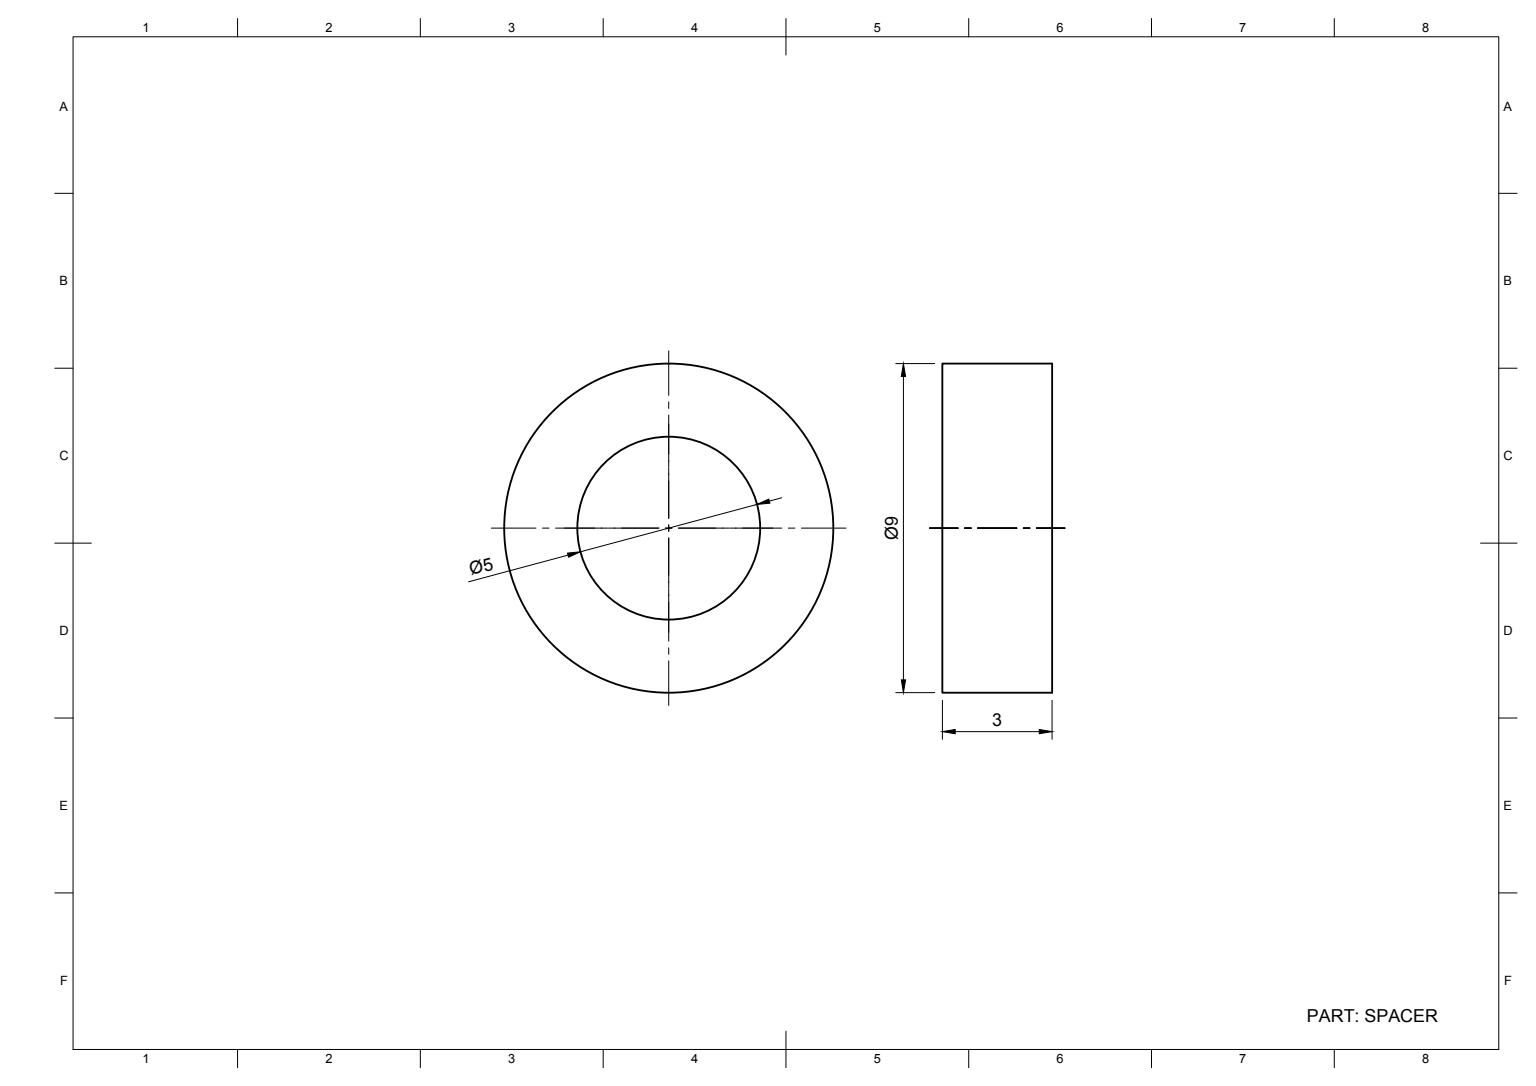
ISO-10303-21;
HEADER;
/* Generated by software containing ST-Developer
 * from STEP Tools, Inc. (www.steptools.com) 
 */

FILE_DESCRIPTION(
/* description */ (''),
/* implementation_level */ '2;1');

FILE_NAME(
/* name */ 'Spacer.step',
/* time_stamp */ '2026-09-20T21:52:48+06:00',
/* author */ (''),
/* organization */ (''),
/* preprocessor_version */ 'ST-DEVELOPER v20.2',
/* originating_system */ 'Autodesk Translation Framework v15.15.0.0',
/* authorisation */ '');

FILE_SCHEMA (('AUTOMOTIVE_DESIGN { 1 0 10303 214 3 1 1 }'));
ENDSEC;

DATA;
#10=MECHANICAL_DESIGN_GEOMETRIC_PRESENTATION_REPRESENTATION('',(#66),#2203);
#50=SHAPE_REPRESENTATION_RELATIONSHIP('SRR','None',#2242,#58);
#58=ADVANCED_BREP_SHAPE_REPRESENTATION('',(#74),#2202);
#66=STYLED_ITEM('',(#2286),#74);
#74=MANIFOLD_SOLID_BREP('Spacer',#1233);
#87=FACE_BOUND('',#308,.T.);
#88=FACE_BOUND('',#312,.T.);
#133=CIRCLE('',#1442,4.5);
#134=CIRCLE('',#1443,2.5);
#135=CIRCLE('',#1445,4.5);
#136=CIRCLE('',#1447,2.5);
#159=CYLINDRICAL_SURFACE('',#1444,4.5);
#160=CYLINDRICAL_SURFACE('',#1446,2.5);
#226=FACE_OUTER_BOUND('',#307,.T.);
#227=FACE_OUTER_BOUND('',#309,.T.);
#228=FACE_OUTER_BOUND('',#310,.T.);
#229=FACE_OUTER_BOUND('',#311,.T.);
#307=EDGE_LOOP('',(#1100));
#308=EDGE_LOOP('',(#1101));
#309=EDGE_LOOP('',(#1102,#1103,#1104,#1105));
#310=EDGE_LOOP('',(#1106,#1107,#1108,#1109));
#311=EDGE_LOOP('',(#1110));
#312=EDGE_LOOP('',(#1111));
#421=LINE('',#2169,#531);
#422=LINE('',#2174,#532);
#531=VECTOR('',#1809,4.5);
#532=VECTOR('',#1816,2.5);
#634=VERTEX_POINT('',#2163);
#635=VERTEX_POINT('',#2165);
#636=VERTEX_POINT('',#2168);
#637=VERTEX_POINT('',#2172);
#790=EDGE_CURVE('',#634,#634,#133,.T.);
#791=EDGE_CURVE('',#635,#635,#134,.T.);
#792=EDGE_CURVE('',#634,#636,#421,.T.);
#793=EDGE_CURVE('',#636,#636,#135,.T.);
#794=EDGE_CURVE('',#637,#637,#136,.T.);
#795=EDGE_CURVE('',#637,#635,#422,.T.);
#1100=ORIENTED_EDGE('',*,*,#790,.T.);
#1101=ORIENTED_EDGE('',*,*,#791,.T.);
#1102=ORIENTED_EDGE('',*,*,#790,.F.);
#1103=ORIENTED_EDGE('',*,*,#792,.T.);
#1104=ORIENTED_EDGE('',*,*,#793,.F.);
#1105=ORIENTED_EDGE('',*,*,#792,.F.);
#1106=ORIENTED_EDGE('',*,*,#794,.F.);
#1107=ORIENTED_EDGE('',*,*,#795,.T.);
#1108=ORIENTED_EDGE('',*,*,#791,.F.);
#1109=ORIENTED_EDGE('',*,*,#795,.F.);
#1110=ORIENTED_EDGE('',*,*,#793,.T.);
#1111=ORIENTED_EDGE('',*,*,#794,.T.);
#1155=PLANE('',#1441);
#1156=PLANE('',#1448);
#1222=ADVANCED_FACE('',(#226,#87),#1155,.T.);
#1223=ADVANCED_FACE('',(#227),#159,.T.);
#1224=ADVANCED_FACE('',(#228),#160,.F.);
#1225=ADVANCED_FACE('',(#229,#88),#1156,.T.);
#1233=CLOSED_SHELL('',(#1222,#1223,#1224,#1225));
#1440=AXIS2_PLACEMENT_3D('',#2161,#1799,#1800);
#1441=AXIS2_PLACEMENT_3D('',#2162,#1801,#1802);
#1442=AXIS2_PLACEMENT_3D('',#2164,#1803,#1804);
#1443=AXIS2_PLACEMENT_3D('',#2166,#1805,#1806);
#1444=AXIS2_PLACEMENT_3D('',#2167,#1807,#1808);
#1445=AXIS2_PLACEMENT_3D('',#2170,#1810,#1811);
#1446=AXIS2_PLACEMENT_3D('',#2171,#1812,#1813);
#1447=AXIS2_PLACEMENT_3D('',#2173,#1814,#1815);
#1448=AXIS2_PLACEMENT_3D('',#2175,#1817,#1818);
#1799=DIRECTION('axis',(0.,0.,1.));
#1800=DIRECTION('refdir',(1.,0.,0.));
#1801=DIRECTION('center_axis',(0.,-1.,0.));
#1802=DIRECTION('ref_axis',(1.,0.,0.));
#1803=DIRECTION('center_axis',(0.,-1.,0.));
#1804=DIRECTION('ref_axis',(1.,0.,0.));
#1805=DIRECTION('center_axis',(0.,1.,0.));
#1806=DIRECTION('ref_axis',(1.,0.,0.));
#1807=DIRECTION('center_axis',(0.,-1.,0.));
#1808=DIRECTION('ref_axis',(1.,0.,0.));
#1809=DIRECTION('',(0.,1.,0.));
#1810=DIRECTION('center_axis',(0.,1.,0.));
#1811=DIRECTION('ref_axis',(1.,0.,0.));
#1812=DIRECTION('center_axis',(0.,-1.,0.));
#1813=DIRECTION('ref_axis',(1.,0.,0.));
#1814=DIRECTION('center_axis',(0.,-1.,0.));
#1815=DIRECTION('ref_axis',(1.,0.,0.));
#1816=DIRECTION('',(0.,-1.,0.));
#1817=DIRECTION('center_axis',(0.,1.,0.));
#1818=DIRECTION('ref_axis',(0.,0.,1.));
#2161=CARTESIAN_POINT('',(0.,0.,0.));
#2162=CARTESIAN_POINT('Origin',(1.66533453693773E-15,0.,72.8759738016714));
#2163=CARTESIAN_POINT('',(-4.5,0.,72.8759738016714));
#2164=CARTESIAN_POINT('Origin',(1.53080849893419E-15,0.,72.8759738016714));
#2165=CARTESIAN_POINT('',(-2.5,0.,72.8759738016714));
#2166=CARTESIAN_POINT('Origin',(1.53080849893419E-15,0.,72.8759738016714));
#2167=CARTESIAN_POINT('Origin',(1.53080849893419E-15,3.,72.8759738016714));
#2168=CARTESIAN_POINT('',(-4.5,3.,72.8759738016714));
#2169=CARTESIAN_POINT('',(-4.5,3.,72.8759738016714));
#2170=CARTESIAN_POINT('Origin',(1.53080849893419E-15,3.,72.8759738016714));
#2171=CARTESIAN_POINT('Origin',(1.53080849893419E-15,3.,72.8759738016714));
#2172=CARTESIAN_POINT('',(-2.5,3.,72.8759738016714));
#2173=CARTESIAN_POINT('Origin',(1.53080849893419E-15,3.,72.8759738016714));
#2174=CARTESIAN_POINT('',(-2.5,3.,72.8759738016714));
#2175=CARTESIAN_POINT('Origin',(0.,3.,50.));
#2192=UNCERTAINTY_MEASURE_WITH_UNIT(LENGTH_MEASURE(0.01),#2204,
'DISTANCE_ACCURACY_VALUE',
'Maximum model space distance between geometric entities at asserted c
onnectivities');
#2193=UNCERTAINTY_MEASURE_WITH_UNIT(LENGTH_MEASURE(0.01),#2204,
'DISTANCE_ACCURACY_VALUE',
'Maximum model space distance between geometric entities at asserted c
onnectivities');
#2202=(
GEOMETRIC_REPRESENTATION_CONTEXT(3)
GLOBAL_UNCERTAINTY_ASSIGNED_CONTEXT((#2192))
GLOBAL_UNIT_ASSIGNED_CONTEXT((#2204,#2206,#2207))
REPRESENTATION_CONTEXT('','3D')
);
#2203=(
GEOMETRIC_REPRESENTATION_CONTEXT(3)
GLOBAL_UNCERTAINTY_ASSIGNED_CONTEXT((#2193))
GLOBAL_UNIT_ASSIGNED_CONTEXT((#2204,#2206,#2207))
REPRESENTATION_CONTEXT('','3D')
);
#2204=(
LENGTH_UNIT()
NAMED_UNIT(*)
SI_UNIT(.MILLI.,.METRE.)
);
#2206=(
NAMED_UNIT(*)
PLANE_ANGLE_UNIT()
SI_UNIT($,.RADIAN.)
);
#2207=(
NAMED_UNIT(*)
SI_UNIT($,.STERADIAN.)
SOLID_ANGLE_UNIT()
);
#2216=SHAPE_DEFINITION_REPRESENTATION(#2225,#2242);
#2225=PRODUCT_DEFINITION_SHAPE('',$,#2252);
#2242=SHAPE_REPRESENTATION('',(#1440),#2202);
#2243=PRODUCT_DEFINITION_CONTEXT('part definition',#2272,'design');
#2252=PRODUCT_DEFINITION('Spacer','Spacer',#2261,#2243);
#2261=PRODUCT_DEFINITION_FORMATION('',$,#2282);
#2272=APPLICATION_CONTEXT(
'Core Data for Automotive Mechanical Design Process');
#2273=PRODUCT_CONTEXT('part definition',#2272,'mechanical');
#2282=PRODUCT('Spacer','Spacer',$,(#2273));
#2286=PRESENTATION_STYLE_ASSIGNMENT((#2290));
#2290=SURFACE_STYLE_USAGE(.BOTH.,#2294);
#2294=SURFACE_SIDE_STYLE('',(#2298));
#2298=SURFACE_STYLE_FILL_AREA(#2302);
#2302=FILL_AREA_STYLE('Surface - Matte',(#2306));
#2306=FILL_AREA_STYLE_COLOUR('Surface - Matte',#2310);
#2310=COLOUR_RGB('Surface - Matte', 0.31764706, 0.68627451, 0.89019608);
ENDSEC;
END-ISO-10303-21;
